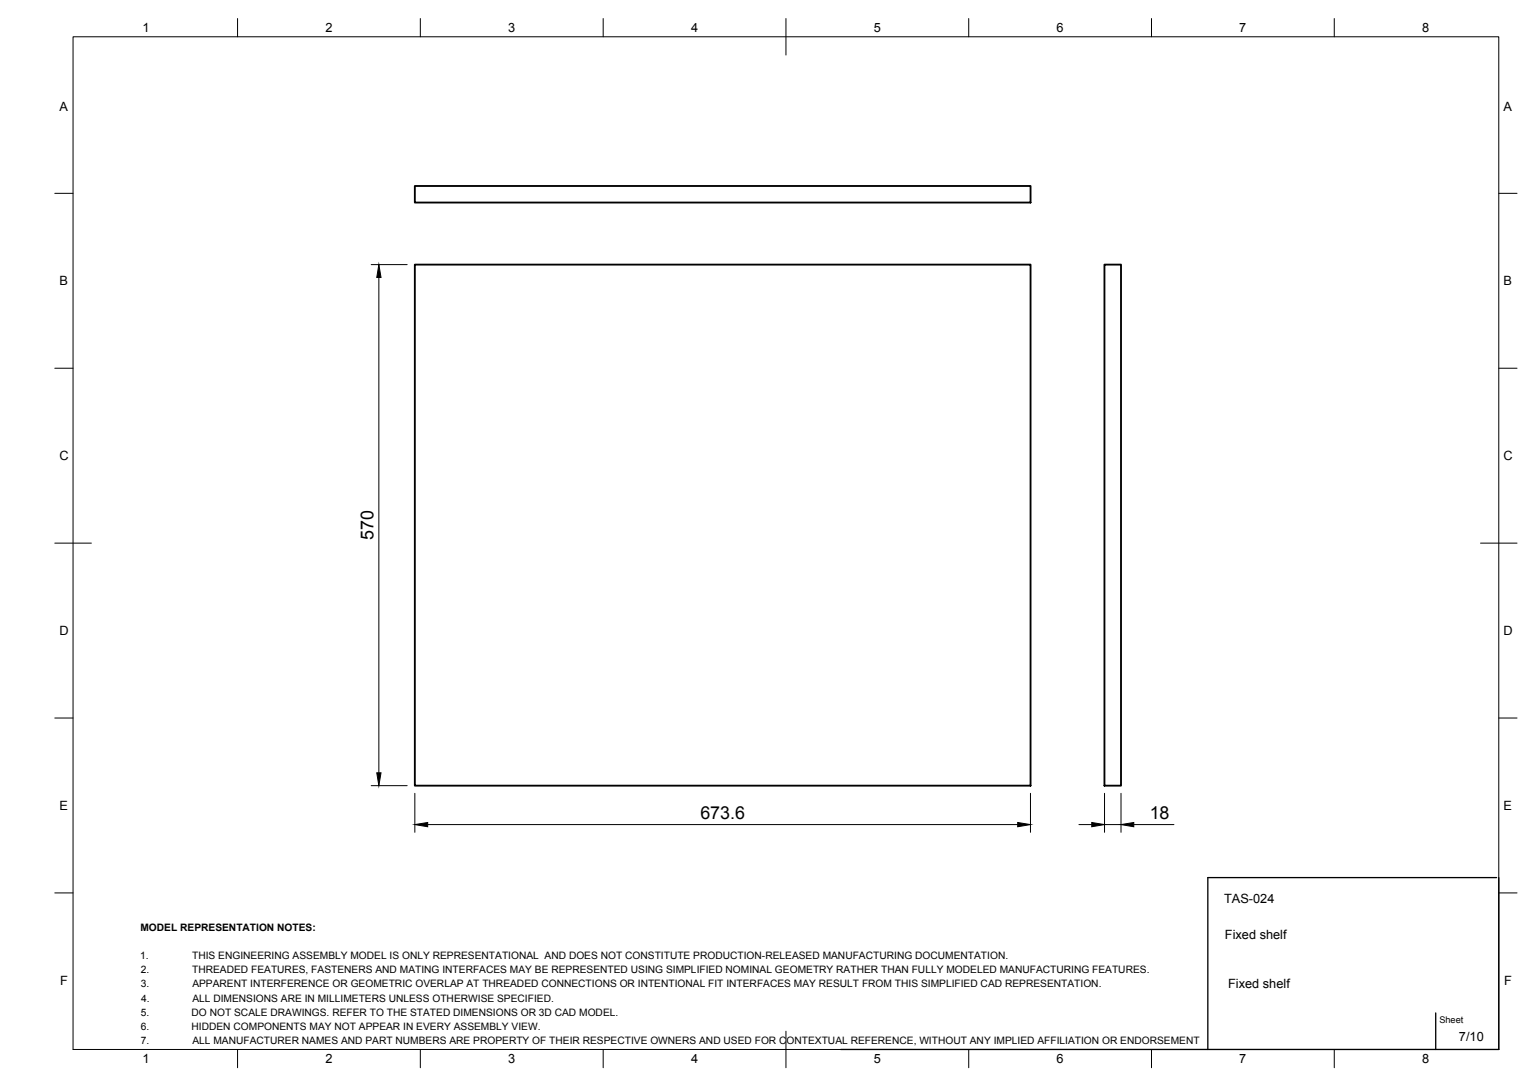
ISO-10303-21;
HEADER;
/* Generated by software containing ST-Developer
 * from STEP Tools, Inc. (www.steptools.com) 
 */

FILE_DESCRIPTION(
/* description */ (''),
/* implementation_level */ '2;1');

FILE_NAME(
/* name */ 'Fixed shelf.step',
/* time_stamp */ '2026-11-15T17:53:25-08:00',
/* author */ (''),
/* organization */ (''),
/* preprocessor_version */ 'ST-DEVELOPER v20.2',
/* originating_system */ 'Autodesk Translation Framework v15.17.0.0',
/* authorisation */ '');

FILE_SCHEMA (('AUTOMOTIVE_DESIGN { 1 0 10303 214 3 1 1 }'));
ENDSEC;

DATA;
#10=MECHANICAL_DESIGN_GEOMETRIC_PRESENTATION_REPRESENTATION('',(#135),#2673);
#119=SHAPE_REPRESENTATION_RELATIONSHIP('SRR','None',#2727,#127);
#127=ADVANCED_BREP_SHAPE_REPRESENTATION('',(#143),#2669);
#135=STYLED_ITEM('',(#2776),#143);
#143=MANIFOLD_SOLID_BREP('Body1',#1521);
#218=PLANE('',#1708);
#219=PLANE('',#1709);
#220=PLANE('',#1710);
#221=PLANE('',#1711);
#222=PLANE('',#1712);
#223=PLANE('',#1713);
#301=FACE_OUTER_BOUND('',#400,.T.);
#302=FACE_OUTER_BOUND('',#401,.T.);
#303=FACE_OUTER_BOUND('',#402,.T.);
#304=FACE_OUTER_BOUND('',#403,.T.);
#305=FACE_OUTER_BOUND('',#404,.T.);
#306=FACE_OUTER_BOUND('',#405,.T.);
#400=EDGE_LOOP('',(#1352,#1353,#1354,#1355));
#401=EDGE_LOOP('',(#1356,#1357,#1358,#1359));
#402=EDGE_LOOP('',(#1360,#1361,#1362,#1363));
#403=EDGE_LOOP('',(#1364,#1365,#1366,#1367));
#404=EDGE_LOOP('',(#1368,#1369,#1370,#1371));
#405=EDGE_LOOP('',(#1372,#1373,#1374,#1375));
#554=LINE('',#2557,#702);
#555=LINE('',#2559,#703);
#556=LINE('',#2561,#704);
#557=LINE('',#2562,#705);
#558=LINE('',#2565,#706);
#559=LINE('',#2567,#707);
#560=LINE('',#2568,#708);
#561=LINE('',#2571,#709);
#562=LINE('',#2573,#710);
#563=LINE('',#2574,#711);
#564=LINE('',#2576,#712);
#565=LINE('',#2577,#713);
#702=VECTOR('',#2090,1.);
#703=VECTOR('',#2091,1.);
#704=VECTOR('',#2092,1.);
#705=VECTOR('',#2093,1.);
#706=VECTOR('',#2096,1.);
#707=VECTOR('',#2097,1.);
#708=VECTOR('',#2098,1.);
#709=VECTOR('',#2101,1.);
#710=VECTOR('',#2102,1.);
#711=VECTOR('',#2103,1.);
#712=VECTOR('',#2106,1.);
#713=VECTOR('',#2107,1.);
#852=VERTEX_POINT('',#2555);
#853=VERTEX_POINT('',#2556);
#854=VERTEX_POINT('',#2558);
#855=VERTEX_POINT('',#2560);
#856=VERTEX_POINT('',#2564);
#857=VERTEX_POINT('',#2566);
#858=VERTEX_POINT('',#2570);
#859=VERTEX_POINT('',#2572);
#1022=EDGE_CURVE('',#852,#853,#554,.T.);
#1023=EDGE_CURVE('',#853,#854,#555,.T.);
#1024=EDGE_CURVE('',#855,#854,#556,.T.);
#1025=EDGE_CURVE('',#852,#855,#557,.T.);
#1026=EDGE_CURVE('',#856,#852,#558,.T.);
#1027=EDGE_CURVE('',#857,#855,#559,.T.);
#1028=EDGE_CURVE('',#856,#857,#560,.T.);
#1029=EDGE_CURVE('',#858,#856,#561,.T.);
#1030=EDGE_CURVE('',#859,#857,#562,.T.);
#1031=EDGE_CURVE('',#858,#859,#563,.T.);
#1032=EDGE_CURVE('',#853,#858,#564,.T.);
#1033=EDGE_CURVE('',#854,#859,#565,.T.);
#1352=ORIENTED_EDGE('',*,*,#1022,.T.);
#1353=ORIENTED_EDGE('',*,*,#1023,.T.);
#1354=ORIENTED_EDGE('',*,*,#1024,.F.);
#1355=ORIENTED_EDGE('',*,*,#1025,.F.);
#1356=ORIENTED_EDGE('',*,*,#1026,.T.);
#1357=ORIENTED_EDGE('',*,*,#1025,.T.);
#1358=ORIENTED_EDGE('',*,*,#1027,.F.);
#1359=ORIENTED_EDGE('',*,*,#1028,.F.);
#1360=ORIENTED_EDGE('',*,*,#1029,.T.);
#1361=ORIENTED_EDGE('',*,*,#1028,.T.);
#1362=ORIENTED_EDGE('',*,*,#1030,.F.);
#1363=ORIENTED_EDGE('',*,*,#1031,.F.);
#1364=ORIENTED_EDGE('',*,*,#1032,.T.);
#1365=ORIENTED_EDGE('',*,*,#1031,.T.);
#1366=ORIENTED_EDGE('',*,*,#1033,.F.);
#1367=ORIENTED_EDGE('',*,*,#1023,.F.);
#1368=ORIENTED_EDGE('',*,*,#1033,.T.);
#1369=ORIENTED_EDGE('',*,*,#1030,.T.);
#1370=ORIENTED_EDGE('',*,*,#1027,.T.);
#1371=ORIENTED_EDGE('',*,*,#1024,.T.);
#1372=ORIENTED_EDGE('',*,*,#1032,.F.);
#1373=ORIENTED_EDGE('',*,*,#1022,.F.);
#1374=ORIENTED_EDGE('',*,*,#1026,.F.);
#1375=ORIENTED_EDGE('',*,*,#1029,.F.);
#1496=ADVANCED_FACE('',(#301),#218,.T.);
#1497=ADVANCED_FACE('',(#302),#219,.T.);
#1498=ADVANCED_FACE('',(#303),#220,.T.);
#1499=ADVANCED_FACE('',(#304),#221,.T.);
#1500=ADVANCED_FACE('',(#305),#222,.T.);
#1501=ADVANCED_FACE('',(#306),#223,.F.);
#1521=CLOSED_SHELL('',(#1496,#1497,#1498,#1499,#1500,#1501));
#1707=AXIS2_PLACEMENT_3D('',#2553,#2086,#2087);
#1708=AXIS2_PLACEMENT_3D('',#2554,#2088,#2089);
#1709=AXIS2_PLACEMENT_3D('',#2563,#2094,#2095);
#1710=AXIS2_PLACEMENT_3D('',#2569,#2099,#2100);
#1711=AXIS2_PLACEMENT_3D('',#2575,#2104,#2105);
#1712=AXIS2_PLACEMENT_3D('',#2578,#2108,#2109);
#1713=AXIS2_PLACEMENT_3D('',#2579,#2110,#2111);
#2086=DIRECTION('axis',(0.,0.,1.));
#2087=DIRECTION('refdir',(1.,0.,0.));
#2088=DIRECTION('center_axis',(0.,1.,0.));
#2089=DIRECTION('ref_axis',(-1.,0.,0.));
#2090=DIRECTION('',(-1.,0.,0.));
#2091=DIRECTION('',(0.,0.,1.));
#2092=DIRECTION('',(-1.,0.,0.));
#2093=DIRECTION('',(0.,0.,1.));
#2094=DIRECTION('center_axis',(1.,0.,0.));
#2095=DIRECTION('ref_axis',(0.,1.,0.));
#2096=DIRECTION('',(0.,1.,0.));
#2097=DIRECTION('',(0.,1.,0.));
#2098=DIRECTION('',(0.,0.,1.));
#2099=DIRECTION('center_axis',(0.,-1.,0.));
#2100=DIRECTION('ref_axis',(1.,0.,0.));
#2101=DIRECTION('',(1.,0.,0.));
#2102=DIRECTION('',(1.,0.,0.));
#2103=DIRECTION('',(0.,0.,1.));
#2104=DIRECTION('center_axis',(-1.,0.,0.));
#2105=DIRECTION('ref_axis',(0.,-1.,0.));
#2106=DIRECTION('',(0.,-1.,0.));
#2107=DIRECTION('',(0.,-1.,0.));
#2108=DIRECTION('center_axis',(0.,0.,1.));
#2109=DIRECTION('ref_axis',(1.,0.,0.));
#2110=DIRECTION('center_axis',(0.,0.,1.));
#2111=DIRECTION('ref_axis',(1.,0.,0.));
#2553=CARTESIAN_POINT('',(0.,0.,0.));
#2554=CARTESIAN_POINT('Origin',(67.36,57.6,0.));
#2555=CARTESIAN_POINT('',(67.36,57.6,0.));
#2556=CARTESIAN_POINT('',(0.,57.6,0.));
#2557=CARTESIAN_POINT('',(67.36,57.6,0.));
#2558=CARTESIAN_POINT('',(0.,57.6,1.8));
#2559=CARTESIAN_POINT('',(0.,57.6,0.));
#2560=CARTESIAN_POINT('',(67.36,57.6,1.8));
#2561=CARTESIAN_POINT('',(67.36,57.6,1.8));
#2562=CARTESIAN_POINT('',(67.36,57.6,0.));
#2563=CARTESIAN_POINT('Origin',(67.36,0.6,0.));
#2564=CARTESIAN_POINT('',(67.36,0.6,0.));
#2565=CARTESIAN_POINT('',(67.36,0.6,0.));
#2566=CARTESIAN_POINT('',(67.36,0.600000000000001,1.8));
#2567=CARTESIAN_POINT('',(67.36,0.6,1.8));
#2568=CARTESIAN_POINT('',(67.36,0.6,0.));
#2569=CARTESIAN_POINT('Origin',(0.,0.6,0.));
#2570=CARTESIAN_POINT('',(0.,0.600000000000001,0.));
#2571=CARTESIAN_POINT('',(0.,0.6,0.));
#2572=CARTESIAN_POINT('',(0.,0.600000000000001,1.8));
#2573=CARTESIAN_POINT('',(0.,0.6,1.8));
#2574=CARTESIAN_POINT('',(0.,0.600000000000001,0.));
#2575=CARTESIAN_POINT('Origin',(0.,57.6,0.));
#2576=CARTESIAN_POINT('',(0.,57.6,0.));
#2577=CARTESIAN_POINT('',(0.,57.6,1.8));
#2578=CARTESIAN_POINT('Origin',(33.68,29.1,1.8));
#2579=CARTESIAN_POINT('Origin',(33.68,29.1,0.));
#2659=UNCERTAINTY_MEASURE_WITH_UNIT(LENGTH_MEASURE(0.001),#2674,
'DISTANCE_ACCURACY_VALUE',
'Maximum model space distance between geometric entities at asserted c
onnectivities');
#2663=UNCERTAINTY_MEASURE_WITH_UNIT(LENGTH_MEASURE(0.001),#2674,
'DISTANCE_ACCURACY_VALUE',
'Maximum model space distance between geometric entities at asserted c
onnectivities');
#2669=(
GEOMETRIC_REPRESENTATION_CONTEXT(3)
GLOBAL_UNCERTAINTY_ASSIGNED_CONTEXT((#2659))
GLOBAL_UNIT_ASSIGNED_CONTEXT((#2674,#2676,#2677))
REPRESENTATION_CONTEXT('','3D')
);
#2673=(
GEOMETRIC_REPRESENTATION_CONTEXT(3)
GLOBAL_UNCERTAINTY_ASSIGNED_CONTEXT((#2663))
GLOBAL_UNIT_ASSIGNED_CONTEXT((#2674,#2676,#2677))
REPRESENTATION_CONTEXT('','3D')
);
#2674=(
LENGTH_UNIT()
NAMED_UNIT(*)
SI_UNIT(.CENTI.,.METRE.)
);
#2676=(
NAMED_UNIT(*)
PLANE_ANGLE_UNIT()
SI_UNIT($,.RADIAN.)
);
#2677=(
NAMED_UNIT(*)
SI_UNIT($,.STERADIAN.)
SOLID_ANGLE_UNIT()
);
#2683=SHAPE_DEFINITION_REPRESENTATION(#2692,#2727);
#2692=PRODUCT_DEFINITION_SHAPE('',$,#2737);
#2727=SHAPE_REPRESENTATION('',(#1707),#2669);
#2731=PRODUCT_DEFINITION_CONTEXT('part definition',#2760,'design');
#2737=PRODUCT_DEFINITION('Fixed shelf','Fixed shelf',#2746,#2731);
#2746=PRODUCT_DEFINITION_FORMATION('',$,#2767);
#2760=APPLICATION_CONTEXT(
'Core Data for Automotive Mechanical Design Process');
#2761=PRODUCT_CONTEXT('part definition',#2760,'mechanical');
#2767=PRODUCT('Fixed shelf','Fixed shelf',$,(#2761));
#2776=PRESENTATION_STYLE_ASSIGNMENT((#2785));
#2785=SURFACE_STYLE_USAGE(.BOTH.,#2794);
#2794=SURFACE_SIDE_STYLE('',(#2803));
#2803=SURFACE_STYLE_FILL_AREA(#2812);
#2812=FILL_AREA_STYLE('Fixed shelf finish',(#2821));
#2821=FILL_AREA_STYLE_COLOUR('Fixed shelf finish',#2830);
#2830=COLOUR_RGB('Fixed shelf finish',0.274509803921569,0.6,0.8);
ENDSEC;
END-ISO-10303-21;
